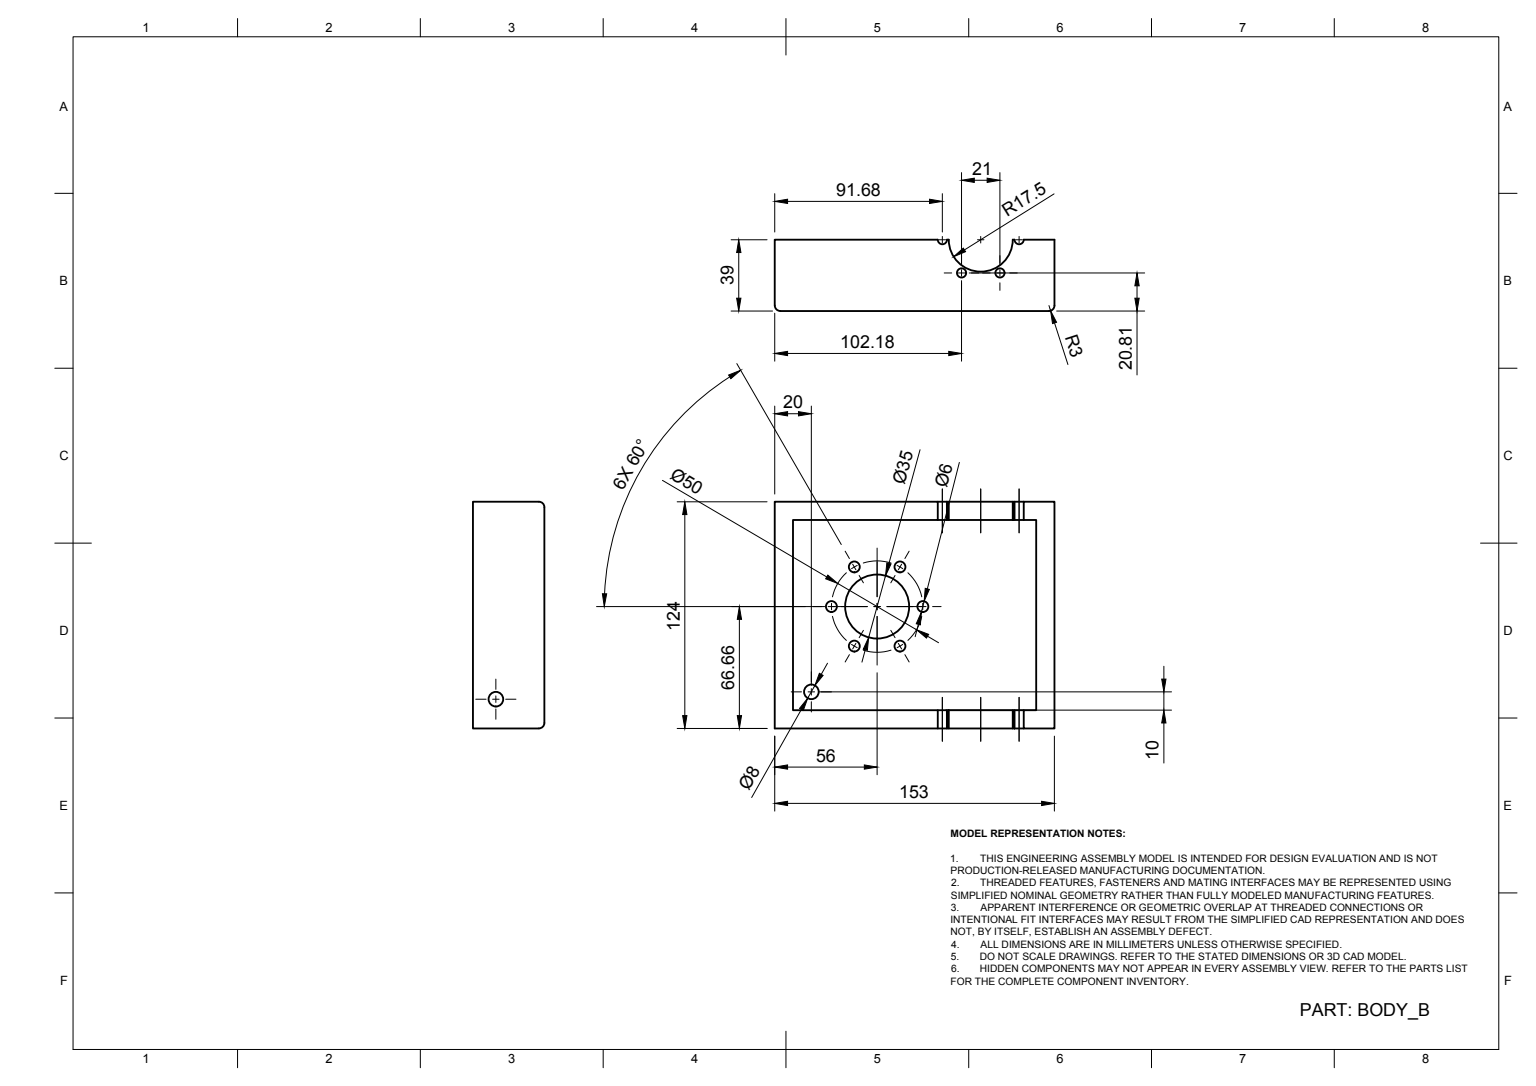
ISO-10303-21;
HEADER;
/* Generated by software containing ST-Developer
 * from STEP Tools, Inc. (www.steptools.com) 
 */

FILE_DESCRIPTION(
/* description */ ('STEP AP214'),
/* implementation_level */ '2;1');

FILE_NAME(
/* name */ 'Body_B.step',
/* time_stamp */ '2026-10-05T13:15:56-07:00',
/* author */ (''),
/* organization */ (''),
/* preprocessor_version */ 'ST-DEVELOPER v20.2',
/* originating_system */ 'Autodesk Translation Framework v15.15.0.0',
/* authorisation */ '');

FILE_SCHEMA (('AUTOMOTIVE_DESIGN { 1 0 10303 214 3 1 1 }'));
ENDSEC;

DATA;
#10=MECHANICAL_DESIGN_GEOMETRIC_PRESENTATION_REPRESENTATION('',(#1349),#37881);
#1325=SHAPE_REPRESENTATION_RELATIONSHIP('SRR','None',#37958,#1337);
#1337=ADVANCED_BREP_SHAPE_REPRESENTATION('',(#1361),#37873);
#1349=STYLED_ITEM('',(#38023),#1361);
#1361=MANIFOLD_SOLID_BREP('Body1',#10823);
#1373=ELLIPSE('',#11682,4.24264068711892,2.99999999999971);
#1374=ELLIPSE('',#11683,4.24264068711757,2.99999999999883);
#1375=ELLIPSE('',#11685,4.24264068711876,2.99999999999963);
#1376=ELLIPSE('',#11687,4.24264068711788,2.99999999999899);
#1407=FACE_BOUND('',#2710,.T.);
#1408=FACE_BOUND('',#2711,.T.);
#1409=FACE_BOUND('',#2714,.T.);
#1410=FACE_BOUND('',#2715,.T.);
#1411=FACE_BOUND('',#2718,.T.);
#1412=FACE_BOUND('',#2720,.T.);
#1413=FACE_BOUND('',#2721,.T.);
#1414=FACE_BOUND('',#2723,.T.);
#1415=FACE_BOUND('',#2725,.T.);
#1416=FACE_BOUND('',#2726,.T.);
#1417=FACE_BOUND('',#2729,.T.);
#1418=FACE_BOUND('',#2730,.T.);
#1419=FACE_BOUND('',#2731,.T.);
#1420=FACE_BOUND('',#2732,.T.);
#1421=FACE_BOUND('',#2733,.T.);
#1422=FACE_BOUND('',#2734,.T.);
#1423=FACE_BOUND('',#2735,.T.);
#1424=FACE_BOUND('',#2736,.T.);
#1425=FACE_BOUND('',#2738,.T.);
#1426=FACE_BOUND('',#2739,.T.);
#1427=FACE_BOUND('',#2740,.T.);
#1428=FACE_BOUND('',#2741,.T.);
#1429=FACE_BOUND('',#2742,.T.);
#1430=FACE_BOUND('',#2743,.T.);
#1431=FACE_BOUND('',#2744,.T.);
#1432=FACE_BOUND('',#2745,.T.);
#1509=PLANE('',#11647);
#1510=PLANE('',#11648);
#1511=PLANE('',#11649);
#1512=PLANE('',#11650);
#1513=PLANE('',#11651);
#1514=PLANE('',#11652);
#1515=PLANE('',#11656);
#1516=PLANE('',#11657);
#1517=PLANE('',#11661);
#1518=PLANE('',#11662);
#1519=PLANE('',#11663);
#1520=PLANE('',#11667);
#1521=PLANE('',#11668);
#1522=PLANE('',#11672);
#1523=PLANE('',#11673);
#1524=PLANE('',#11674);
#2052=FACE_OUTER_BOUND('',#2691,.T.);
#2053=FACE_OUTER_BOUND('',#2692,.T.);
#2054=FACE_OUTER_BOUND('',#2693,.T.);
#2055=FACE_OUTER_BOUND('',#2694,.T.);
#2056=FACE_OUTER_BOUND('',#2695,.T.);
#2057=FACE_OUTER_BOUND('',#2696,.T.);
#2058=FACE_OUTER_BOUND('',#2697,.T.);
#2059=FACE_OUTER_BOUND('',#2698,.T.);
#2060=FACE_OUTER_BOUND('',#2699,.T.);
#2061=FACE_OUTER_BOUND('',#2700,.T.);
#2062=FACE_OUTER_BOUND('',#2701,.T.);
#2063=FACE_OUTER_BOUND('',#2702,.T.);
#2064=FACE_OUTER_BOUND('',#2703,.T.);
#2065=FACE_OUTER_BOUND('',#2704,.T.);
#2066=FACE_OUTER_BOUND('',#2705,.T.);
#2067=FACE_OUTER_BOUND('',#2706,.T.);
#2068=FACE_OUTER_BOUND('',#2707,.T.);
#2069=FACE_OUTER_BOUND('',#2708,.T.);
#2070=FACE_OUTER_BOUND('',#2709,.T.);
#2071=FACE_OUTER_BOUND('',#2712,.T.);
#2072=FACE_OUTER_BOUND('',#2713,.T.);
#2073=FACE_OUTER_BOUND('',#2716,.T.);
#2074=FACE_OUTER_BOUND('',#2717,.T.);
#2075=FACE_OUTER_BOUND('',#2719,.T.);
#2076=FACE_OUTER_BOUND('',#2722,.T.);
#2077=FACE_OUTER_BOUND('',#2724,.T.);
#2078=FACE_OUTER_BOUND('',#2727,.T.);
#2079=FACE_OUTER_BOUND('',#2728,.T.);
#2080=FACE_OUTER_BOUND('',#2737,.T.);
#2081=FACE_OUTER_BOUND('',#2746,.T.);
#2082=FACE_OUTER_BOUND('',#2747,.T.);
#2083=FACE_OUTER_BOUND('',#2748,.T.);
#2084=FACE_OUTER_BOUND('',#2749,.T.);
#2085=FACE_OUTER_BOUND('',#2750,.T.);
#2086=FACE_OUTER_BOUND('',#2751,.T.);
#2087=FACE_OUTER_BOUND('',#2752,.T.);
#2088=FACE_OUTER_BOUND('',#2753,.T.);
#2089=FACE_OUTER_BOUND('',#2754,.T.);
#2090=FACE_OUTER_BOUND('',#2755,.T.);
#2691=EDGE_LOOP('',(#9463,#9464,#9465,#9466));
#2692=EDGE_LOOP('',(#9467,#9468,#9469,#9470));
#2693=EDGE_LOOP('',(#9471,#9472,#9473,#9474));
#2694=EDGE_LOOP('',(#9475,#9476,#9477,#9478));
#2695=EDGE_LOOP('',(#9479,#9480,#9481,#9482));
#2696=EDGE_LOOP('',(#9483,#9484,#9485,#9486));
#2697=EDGE_LOOP('',(#9487,#9488,#9489,#9490));
#2698=EDGE_LOOP('',(#9491,#9492,#9493,#9494));
#2699=EDGE_LOOP('',(#9495,#9496,#9497,#9498));
#2700=EDGE_LOOP('',(#9499,#9500,#9501,#9502));
#2701=EDGE_LOOP('',(#9503,#9504,#9505,#9506));
#2702=EDGE_LOOP('',(#9507,#9508,#9509,#9510));
#2703=EDGE_LOOP('',(#9511,#9512,#9513,#9514));
#2704=EDGE_LOOP('',(#9515,#9516,#9517,#9518,#9519,#9520,#9521,#9522));
#2705=EDGE_LOOP('',(#9523,#9524,#9525,#9526));
#2706=EDGE_LOOP('',(#9527,#9528,#9529,#9530));
#2707=EDGE_LOOP('',(#9531,#9532,#9533,#9534));
#2708=EDGE_LOOP('',(#9535,#9536,#9537,#9538));
#2709=EDGE_LOOP('',(#9539,#9540,#9541,#9542,#9543,#9544,#9545,#9546,#9547,
#9548));
#2710=EDGE_LOOP('',(#9549));
#2711=EDGE_LOOP('',(#9550));
#2712=EDGE_LOOP('',(#9551,#9552,#9553,#9554,#9555,#9556,#9557,#9558));
#2713=EDGE_LOOP('',(#9559,#9560,#9561,#9562,#9563,#9564,#9565,#9566,#9567,
#9568));
#2714=EDGE_LOOP('',(#9569));
#2715=EDGE_LOOP('',(#9570));
#2716=EDGE_LOOP('',(#9571,#9572,#9573,#9574));
#2717=EDGE_LOOP('',(#9575,#9576,#9577,#9578));
#2718=EDGE_LOOP('',(#9579));
#2719=EDGE_LOOP('',(#9580,#9581,#9582,#9583,#9584,#9585,#9586,#9587,#9588,
#9589));
#2720=EDGE_LOOP('',(#9590));
#2721=EDGE_LOOP('',(#9591));
#2722=EDGE_LOOP('',(#9592,#9593,#9594,#9595));
#2723=EDGE_LOOP('',(#9596));
#2724=EDGE_LOOP('',(#9597,#9598,#9599,#9600,#9601,#9602,#9603,#9604,#9605,
#9606));
#2725=EDGE_LOOP('',(#9607));
#2726=EDGE_LOOP('',(#9608));
#2727=EDGE_LOOP('',(#9609,#9610,#9611,#9612));
#2728=EDGE_LOOP('',(#9613,#9614,#9615,#9616));
#2729=EDGE_LOOP('',(#9617));
#2730=EDGE_LOOP('',(#9618));
#2731=EDGE_LOOP('',(#9619));
#2732=EDGE_LOOP('',(#9620));
#2733=EDGE_LOOP('',(#9621));
#2734=EDGE_LOOP('',(#9622));
#2735=EDGE_LOOP('',(#9623));
#2736=EDGE_LOOP('',(#9624));
#2737=EDGE_LOOP('',(#9625,#9626,#9627,#9628));
#2738=EDGE_LOOP('',(#9629));
#2739=EDGE_LOOP('',(#9630));
#2740=EDGE_LOOP('',(#9631));
#2741=EDGE_LOOP('',(#9632));
#2742=EDGE_LOOP('',(#9633));
#2743=EDGE_LOOP('',(#9634));
#2744=EDGE_LOOP('',(#9635));
#2745=EDGE_LOOP('',(#9636));
#2746=EDGE_LOOP('',(#9637,#9638,#9639,#9640));
#2747=EDGE_LOOP('',(#9641,#9642,#9643,#9644));
#2748=EDGE_LOOP('',(#9645,#9646,#9647,#9648));
#2749=EDGE_LOOP('',(#9649,#9650,#9651,#9652));
#2750=EDGE_LOOP('',(#9653,#9654,#9655,#9656));
#2751=EDGE_LOOP('',(#9657,#9658,#9659,#9660));
#2752=EDGE_LOOP('',(#9661,#9662,#9663,#9664));
#2753=EDGE_LOOP('',(#9665,#9666,#9667,#9668));
#2754=EDGE_LOOP('',(#9669,#9670,#9671,#9672));
#2755=EDGE_LOOP('',(#9673,#9674,#9675,#9676));
#3001=LINE('',#37226,#3302);
#3002=LINE('',#37232,#3303);
#3003=LINE('',#37238,#3304);
#3004=LINE('',#37244,#3305);
#3005=LINE('',#37250,#3306);
#3006=LINE('',#37256,#3307);
#3007=LINE('',#37262,#3308);
#3008=LINE('',#37268,#3309);
#3009=LINE('',#37274,#3310);
#3010=LINE('',#37280,#3311);
#3011=LINE('',#37286,#3312);
#3012=LINE('',#37292,#3313);
#3013=LINE('',#37298,#3314);
#3014=LINE('',#37303,#3315);
#3015=LINE('',#37305,#3316);
#3016=LINE('',#37307,#3317);
#3017=LINE('',#37309,#3318);
#3018=LINE('',#37311,#3319);
#3019=LINE('',#37313,#3320);
#3020=LINE('',#37315,#3321);
#3021=LINE('',#37316,#3322);
#3022=LINE('',#37320,#3323);
#3023=LINE('',#37322,#3324);
#3024=LINE('',#37324,#3325);
#3025=LINE('',#37325,#3326);
#3026=LINE('',#37329,#3327);
#3027=LINE('',#37331,#3328);
#3028=LINE('',#37333,#3329);
#3029=LINE('',#37334,#3330);
#3030=LINE('',#37338,#3331);
#3031=LINE('',#37340,#3332);
#3032=LINE('',#37342,#3333);
#3033=LINE('',#37343,#3334);
#3034=LINE('',#37347,#3335);
#3035=LINE('',#37349,#3336);
#3036=LINE('',#37351,#3337);
#3037=LINE('',#37352,#3338);
#3038=LINE('',#37355,#3339);
#3039=LINE('',#37361,#3340);
#3040=LINE('',#37363,#3341);
#3041=LINE('',#37364,#3342);
#3042=LINE('',#37367,#3343);
#3043=LINE('',#37369,#3344);
#3044=LINE('',#37371,#3345);
#3045=LINE('',#37373,#3346);
#3046=LINE('',#37375,#3347);
#3047=LINE('',#37377,#3348);
#3048=LINE('',#37378,#3349);
#3049=LINE('',#37381,#3350);
#3050=LINE('',#37386,#3351);
#3051=LINE('',#37387,#3352);
#3052=LINE('',#37389,#3353);
#3053=LINE('',#37391,#3354);
#3054=LINE('',#37395,#3355);
#3055=LINE('',#37397,#3356);
#3056=LINE('',#37398,#3357);
#3057=LINE('',#37403,#3358);
#3058=LINE('',#37404,#3359);
#3059=LINE('',#37410,#3360);
#3060=LINE('',#37411,#3361);
#3061=LINE('',#37413,#3362);
#3062=LINE('',#37418,#3363);
#3063=LINE('',#37420,#3364);
#3064=LINE('',#37422,#3365);
#3065=LINE('',#37423,#3366);
#3302=VECTOR('',#13312,4.);
#3303=VECTOR('',#13319,4.);
#3304=VECTOR('',#13326,2.5);
#3305=VECTOR('',#13333,2.5);
#3306=VECTOR('',#13340,2.5);
#3307=VECTOR('',#13347,2.5);
#3308=VECTOR('',#13354,3.);
#3309=VECTOR('',#13361,2.99999999999999);
#3310=VECTOR('',#13368,3.);
#3311=VECTOR('',#13375,3.);
#3312=VECTOR('',#13382,3.);
#3313=VECTOR('',#13389,3.);
#3314=VECTOR('',#13396,17.5);
#3315=VECTOR('',#13401,1000.);
#3316=VECTOR('',#13402,1000.);
#3317=VECTOR('',#13403,1000.);
#3318=VECTOR('',#13404,1000.);
#3319=VECTOR('',#13405,1000.);
#3320=VECTOR('',#13406,1000.);
#3321=VECTOR('',#13407,1000.);
#3322=VECTOR('',#13408,1000.);
#3323=VECTOR('',#13411,1000.);
#3324=VECTOR('',#13412,1000.);
#3325=VECTOR('',#13413,1000.);
#3326=VECTOR('',#13414,1000.);
#3327=VECTOR('',#13417,1000.);
#3328=VECTOR('',#13418,1000.);
#3329=VECTOR('',#13419,1000.);
#3330=VECTOR('',#13420,1000.);
#3331=VECTOR('',#13423,1000.);
#3332=VECTOR('',#13424,1000.);
#3333=VECTOR('',#13425,1000.);
#3334=VECTOR('',#13426,1000.);
#3335=VECTOR('',#13429,1000.);
#3336=VECTOR('',#13430,1000.);
#3337=VECTOR('',#13431,1000.);
#3338=VECTOR('',#13432,1000.);
#3339=VECTOR('',#13435,1000.);
#3340=VECTOR('',#13442,1000.);
#3341=VECTOR('',#13443,1000.);
#3342=VECTOR('',#13444,1000.);
#3343=VECTOR('',#13447,1000.);
#3344=VECTOR('',#13448,1000.);
#3345=VECTOR('',#13449,1000.);
#3346=VECTOR('',#13450,1000.);
#3347=VECTOR('',#13451,1000.);
#3348=VECTOR('',#13452,1000.);
#3349=VECTOR('',#13453,1000.);
#3350=VECTOR('',#13456,1000.);
#3351=VECTOR('',#13463,1000.);
#3352=VECTOR('',#13464,1000.);
#3353=VECTOR('',#13467,1000.);
#3354=VECTOR('',#13470,1000.);
#3355=VECTOR('',#13475,1000.);
#3356=VECTOR('',#13476,1000.);
#3357=VECTOR('',#13477,1000.);
#3358=VECTOR('',#13484,1000.);
#3359=VECTOR('',#13485,1000.);
#3360=VECTOR('',#13494,1000.);
#3361=VECTOR('',#13495,1000.);
#3362=VECTOR('',#13498,1000.);
#3363=VECTOR('',#13503,1000.);
#3364=VECTOR('',#13504,1000.);
#3365=VECTOR('',#13505,1000.);
#3366=VECTOR('',#13506,1000.);
#3890=CIRCLE('',#11609,4.);
#3891=CIRCLE('',#11610,4.);
#3892=CIRCLE('',#11612,4.);
#3893=CIRCLE('',#11613,4.);
#3894=CIRCLE('',#11615,2.5);
#3895=CIRCLE('',#11616,2.5);
#3896=CIRCLE('',#11618,2.5);
#3897=CIRCLE('',#11619,2.5);
#3898=CIRCLE('',#11621,2.5);
#3899=CIRCLE('',#11622,2.5);
#3900=CIRCLE('',#11624,2.5);
#3901=CIRCLE('',#11625,2.5);
#3902=CIRCLE('',#11627,3.);
#3903=CIRCLE('',#11628,3.);
#3904=CIRCLE('',#11630,2.99999999999999);
#3905=CIRCLE('',#11631,2.99999999999999);
#3906=CIRCLE('',#11633,3.);
#3907=CIRCLE('',#11634,3.);
#3908=CIRCLE('',#11636,3.);
#3909=CIRCLE('',#11637,3.);
#3910=CIRCLE('',#11639,3.);
#3911=CIRCLE('',#11640,3.);
#3912=CIRCLE('',#11642,3.);
#3913=CIRCLE('',#11643,3.);
#3914=CIRCLE('',#11645,17.5);
#3915=CIRCLE('',#11646,17.5);
#3916=CIRCLE('',#11653,2.5);
#3917=CIRCLE('',#11654,17.5);
#3918=CIRCLE('',#11655,2.50000000000001);
#3919=CIRCLE('',#11658,2.50000000000001);
#3920=CIRCLE('',#11659,17.5);
#3921=CIRCLE('',#11660,2.5);
#3922=CIRCLE('',#11664,2.5);
#3923=CIRCLE('',#11665,2.50000000000001);
#3924=CIRCLE('',#11666,17.5);
#3925=CIRCLE('',#11669,2.5);
#3926=CIRCLE('',#11670,17.5);
#3927=CIRCLE('',#11671,2.50000000000001);
#4894=VERTEX_POINT('',#37223);
#4895=VERTEX_POINT('',#37225);
#4896=VERTEX_POINT('',#37229);
#4897=VERTEX_POINT('',#37231);
#4898=VERTEX_POINT('',#37235);
#4899=VERTEX_POINT('',#37237);
#4900=VERTEX_POINT('',#37241);
#4901=VERTEX_POINT('',#37243);
#4902=VERTEX_POINT('',#37247);
#4903=VERTEX_POINT('',#37249);
#4904=VERTEX_POINT('',#37253);
#4905=VERTEX_POINT('',#37255);
#4906=VERTEX_POINT('',#37259);
#4907=VERTEX_POINT('',#37261);
#4908=VERTEX_POINT('',#37265);
#4909=VERTEX_POINT('',#37267);
#4910=VERTEX_POINT('',#37271);
#4911=VERTEX_POINT('',#37273);
#4912=VERTEX_POINT('',#37277);
#4913=VERTEX_POINT('',#37279);
#4914=VERTEX_POINT('',#37283);
#4915=VERTEX_POINT('',#37285);
#4916=VERTEX_POINT('',#37289);
#4917=VERTEX_POINT('',#37291);
#4918=VERTEX_POINT('',#37295);
#4919=VERTEX_POINT('',#37297);
#4920=VERTEX_POINT('',#37301);
#4921=VERTEX_POINT('',#37302);
#4922=VERTEX_POINT('',#37304);
#4923=VERTEX_POINT('',#37306);
#4924=VERTEX_POINT('',#37308);
#4925=VERTEX_POINT('',#37310);
#4926=VERTEX_POINT('',#37312);
#4927=VERTEX_POINT('',#37314);
#4928=VERTEX_POINT('',#37318);
#4929=VERTEX_POINT('',#37319);
#4930=VERTEX_POINT('',#37321);
#4931=VERTEX_POINT('',#37323);
#4932=VERTEX_POINT('',#37327);
#4933=VERTEX_POINT('',#37328);
#4934=VERTEX_POINT('',#37330);
#4935=VERTEX_POINT('',#37332);
#4936=VERTEX_POINT('',#37336);
#4937=VERTEX_POINT('',#37337);
#4938=VERTEX_POINT('',#37339);
#4939=VERTEX_POINT('',#37341);
#4940=VERTEX_POINT('',#37345);
#4941=VERTEX_POINT('',#37346);
#4942=VERTEX_POINT('',#37348);
#4943=VERTEX_POINT('',#37350);
#4944=VERTEX_POINT('',#37354);
#4945=VERTEX_POINT('',#37358);
#4946=VERTEX_POINT('',#37360);
#4947=VERTEX_POINT('',#37362);
#4948=VERTEX_POINT('',#37366);
#4949=VERTEX_POINT('',#37368);
#4950=VERTEX_POINT('',#37370);
#4951=VERTEX_POINT('',#37372);
#4952=VERTEX_POINT('',#37374);
#4953=VERTEX_POINT('',#37376);
#4954=VERTEX_POINT('',#37380);
#4955=VERTEX_POINT('',#37385);
#4956=VERTEX_POINT('',#37394);
#4957=VERTEX_POINT('',#37396);
#4958=VERTEX_POINT('',#37402);
#4959=VERTEX_POINT('',#37409);
#4960=VERTEX_POINT('',#37416);
#4961=VERTEX_POINT('',#37417);
#4962=VERTEX_POINT('',#37419);
#4963=VERTEX_POINT('',#37421);
#6442=EDGE_CURVE('',#4894,#4894,#3890,.T.);
#6443=EDGE_CURVE('',#4894,#4895,#3001,.T.);
#6444=EDGE_CURVE('',#4895,#4895,#3891,.T.);
#6445=EDGE_CURVE('',#4896,#4896,#3892,.T.);
#6446=EDGE_CURVE('',#4896,#4897,#3002,.T.);
#6447=EDGE_CURVE('',#4897,#4897,#3893,.T.);
#6448=EDGE_CURVE('',#4898,#4898,#3894,.T.);
#6449=EDGE_CURVE('',#4898,#4899,#3003,.T.);
#6450=EDGE_CURVE('',#4899,#4899,#3895,.T.);
#6451=EDGE_CURVE('',#4900,#4900,#3896,.T.);
#6452=EDGE_CURVE('',#4900,#4901,#3004,.T.);
#6453=EDGE_CURVE('',#4901,#4901,#3897,.T.);
#6454=EDGE_CURVE('',#4902,#4902,#3898,.T.);
#6455=EDGE_CURVE('',#4902,#4903,#3005,.T.);
#6456=EDGE_CURVE('',#4903,#4903,#3899,.T.);
#6457=EDGE_CURVE('',#4904,#4904,#3900,.T.);
#6458=EDGE_CURVE('',#4904,#4905,#3006,.T.);
#6459=EDGE_CURVE('',#4905,#4905,#3901,.T.);
#6460=EDGE_CURVE('',#4906,#4906,#3902,.T.);
#6461=EDGE_CURVE('',#4906,#4907,#3007,.T.);
#6462=EDGE_CURVE('',#4907,#4907,#3903,.T.);
#6463=EDGE_CURVE('',#4908,#4908,#3904,.T.);
#6464=EDGE_CURVE('',#4908,#4909,#3008,.T.);
#6465=EDGE_CURVE('',#4909,#4909,#3905,.T.);
#6466=EDGE_CURVE('',#4910,#4910,#3906,.T.);
#6467=EDGE_CURVE('',#4910,#4911,#3009,.T.);
#6468=EDGE_CURVE('',#4911,#4911,#3907,.T.);
#6469=EDGE_CURVE('',#4912,#4912,#3908,.T.);
#6470=EDGE_CURVE('',#4912,#4913,#3010,.T.);
#6471=EDGE_CURVE('',#4913,#4913,#3909,.T.);
#6472=EDGE_CURVE('',#4914,#4914,#3910,.T.);
#6473=EDGE_CURVE('',#4914,#4915,#3011,.T.);
#6474=EDGE_CURVE('',#4915,#4915,#3911,.T.);
#6475=EDGE_CURVE('',#4916,#4916,#3912,.T.);
#6476=EDGE_CURVE('',#4916,#4917,#3012,.T.);
#6477=EDGE_CURVE('',#4917,#4917,#3913,.T.);
#6478=EDGE_CURVE('',#4918,#4918,#3914,.T.);
#6479=EDGE_CURVE('',#4918,#4919,#3013,.T.);
#6480=EDGE_CURVE('',#4919,#4919,#3915,.T.);
#6481=EDGE_CURVE('',#4920,#4921,#3014,.T.);
#6482=EDGE_CURVE('',#4922,#4921,#3015,.T.);
#6483=EDGE_CURVE('',#4923,#4922,#3016,.T.);
#6484=EDGE_CURVE('',#4924,#4923,#3017,.T.);
#6485=EDGE_CURVE('',#4924,#4925,#3018,.T.);
#6486=EDGE_CURVE('',#4925,#4926,#3019,.T.);
#6487=EDGE_CURVE('',#4926,#4927,#3020,.T.);
#6488=EDGE_CURVE('',#4927,#4920,#3021,.T.);
#6489=EDGE_CURVE('',#4928,#4929,#3022,.T.);
#6490=EDGE_CURVE('',#4930,#4929,#3023,.T.);
#6491=EDGE_CURVE('',#4930,#4931,#3024,.T.);
#6492=EDGE_CURVE('',#4931,#4928,#3025,.T.);
#6493=EDGE_CURVE('',#4932,#4933,#3026,.T.);
#6494=EDGE_CURVE('',#4933,#4934,#3027,.T.);
#6495=EDGE_CURVE('',#4934,#4935,#3028,.T.);
#6496=EDGE_CURVE('',#4932,#4935,#3029,.T.);
#6497=EDGE_CURVE('',#4936,#4937,#3030,.T.);
#6498=EDGE_CURVE('',#4938,#4937,#3031,.T.);
#6499=EDGE_CURVE('',#4938,#4939,#3032,.T.);
#6500=EDGE_CURVE('',#4939,#4936,#3033,.T.);
#6501=EDGE_CURVE('',#4940,#4941,#3034,.T.);
#6502=EDGE_CURVE('',#4941,#4942,#3035,.T.);
#6503=EDGE_CURVE('',#4942,#4943,#3036,.T.);
#6504=EDGE_CURVE('',#4940,#4943,#3037,.T.);
#6505=EDGE_CURVE('',#4944,#4926,#3038,.T.);
#6506=EDGE_CURVE('',#4925,#4928,#3916,.T.);
#6507=EDGE_CURVE('',#4931,#4934,#3917,.T.);
#6508=EDGE_CURVE('',#4933,#4945,#3918,.T.);
#6509=EDGE_CURVE('',#4946,#4945,#3039,.T.);
#6510=EDGE_CURVE('',#4947,#4946,#3040,.T.);
#6511=EDGE_CURVE('',#4944,#4947,#3041,.T.);
#6512=EDGE_CURVE('',#4945,#4948,#3042,.T.);
#6513=EDGE_CURVE('',#4949,#4948,#3043,.T.);
#6514=EDGE_CURVE('',#4950,#4949,#3044,.T.);
#6515=EDGE_CURVE('',#4951,#4950,#3045,.T.);
#6516=EDGE_CURVE('',#4951,#4952,#3046,.T.);
#6517=EDGE_CURVE('',#4952,#4953,#3047,.T.);
#6518=EDGE_CURVE('',#4953,#4946,#3048,.T.);
#6519=EDGE_CURVE('',#4954,#4953,#3049,.T.);
#6520=EDGE_CURVE('',#4936,#4952,#3919,.T.);
#6521=EDGE_CURVE('',#4942,#4939,#3920,.T.);
#6522=EDGE_CURVE('',#4920,#4941,#3921,.T.);
#6523=EDGE_CURVE('',#4955,#4927,#3050,.T.);
#6524=EDGE_CURVE('',#4954,#4955,#3051,.T.);
#6525=EDGE_CURVE('',#4947,#4954,#3052,.T.);
#6526=EDGE_CURVE('',#4955,#4944,#3053,.T.);
#6527=EDGE_CURVE('',#4929,#4924,#3922,.T.);
#6528=EDGE_CURVE('',#4956,#4923,#3054,.T.);
#6529=EDGE_CURVE('',#4957,#4956,#3055,.T.);
#6530=EDGE_CURVE('',#4957,#4949,#3056,.T.);
#6531=EDGE_CURVE('',#4948,#4932,#3923,.T.);
#6532=EDGE_CURVE('',#4935,#4930,#3924,.T.);
#6533=EDGE_CURVE('',#4958,#4922,#3057,.T.);
#6534=EDGE_CURVE('',#4956,#4958,#3058,.T.);
#6535=EDGE_CURVE('',#4921,#4940,#3925,.T.);
#6536=EDGE_CURVE('',#4943,#4938,#3926,.T.);
#6537=EDGE_CURVE('',#4937,#4951,#3927,.T.);
#6538=EDGE_CURVE('',#4959,#4950,#3059,.T.);
#6539=EDGE_CURVE('',#4958,#4959,#3060,.T.);
#6540=EDGE_CURVE('',#4959,#4957,#3061,.T.);
#6541=EDGE_CURVE('',#4960,#4961,#3062,.T.);
#6542=EDGE_CURVE('',#4962,#4960,#3063,.T.);
#6543=EDGE_CURVE('',#4963,#4962,#3064,.T.);
#6544=EDGE_CURVE('',#4961,#4963,#3065,.T.);
#6545=EDGE_CURVE('',#4947,#4962,#1373,.T.);
#6546=EDGE_CURVE('',#4960,#4944,#1374,.T.);
#6547=EDGE_CURVE('',#4961,#4955,#1375,.T.);
#6548=EDGE_CURVE('',#4954,#4963,#1376,.T.);
#9463=ORIENTED_EDGE('',*,*,#6442,.F.);
#9464=ORIENTED_EDGE('',*,*,#6443,.T.);
#9465=ORIENTED_EDGE('',*,*,#6444,.T.);
#9466=ORIENTED_EDGE('',*,*,#6443,.F.);
#9467=ORIENTED_EDGE('',*,*,#6445,.F.);
#9468=ORIENTED_EDGE('',*,*,#6446,.T.);
#9469=ORIENTED_EDGE('',*,*,#6447,.T.);
#9470=ORIENTED_EDGE('',*,*,#6446,.F.);
#9471=ORIENTED_EDGE('',*,*,#6448,.F.);
#9472=ORIENTED_EDGE('',*,*,#6449,.T.);
#9473=ORIENTED_EDGE('',*,*,#6450,.F.);
#9474=ORIENTED_EDGE('',*,*,#6449,.F.);
#9475=ORIENTED_EDGE('',*,*,#6451,.F.);
#9476=ORIENTED_EDGE('',*,*,#6452,.T.);
#9477=ORIENTED_EDGE('',*,*,#6453,.F.);
#9478=ORIENTED_EDGE('',*,*,#6452,.F.);
#9479=ORIENTED_EDGE('',*,*,#6454,.T.);
#9480=ORIENTED_EDGE('',*,*,#6455,.T.);
#9481=ORIENTED_EDGE('',*,*,#6456,.F.);
#9482=ORIENTED_EDGE('',*,*,#6455,.F.);
#9483=ORIENTED_EDGE('',*,*,#6457,.T.);
#9484=ORIENTED_EDGE('',*,*,#6458,.T.);
#9485=ORIENTED_EDGE('',*,*,#6459,.F.);
#9486=ORIENTED_EDGE('',*,*,#6458,.F.);
#9487=ORIENTED_EDGE('',*,*,#6460,.T.);
#9488=ORIENTED_EDGE('',*,*,#6461,.T.);
#9489=ORIENTED_EDGE('',*,*,#6462,.F.);
#9490=ORIENTED_EDGE('',*,*,#6461,.F.);
#9491=ORIENTED_EDGE('',*,*,#6463,.T.);
#9492=ORIENTED_EDGE('',*,*,#6464,.T.);
#9493=ORIENTED_EDGE('',*,*,#6465,.F.);
#9494=ORIENTED_EDGE('',*,*,#6464,.F.);
#9495=ORIENTED_EDGE('',*,*,#6466,.T.);
#9496=ORIENTED_EDGE('',*,*,#6467,.T.);
#9497=ORIENTED_EDGE('',*,*,#6468,.F.);
#9498=ORIENTED_EDGE('',*,*,#6467,.F.);
#9499=ORIENTED_EDGE('',*,*,#6469,.T.);
#9500=ORIENTED_EDGE('',*,*,#6470,.T.);
#9501=ORIENTED_EDGE('',*,*,#6471,.F.);
#9502=ORIENTED_EDGE('',*,*,#6470,.F.);
#9503=ORIENTED_EDGE('',*,*,#6472,.T.);
#9504=ORIENTED_EDGE('',*,*,#6473,.T.);
#9505=ORIENTED_EDGE('',*,*,#6474,.F.);
#9506=ORIENTED_EDGE('',*,*,#6473,.F.);
#9507=ORIENTED_EDGE('',*,*,#6475,.T.);
#9508=ORIENTED_EDGE('',*,*,#6476,.T.);
#9509=ORIENTED_EDGE('',*,*,#6477,.F.);
#9510=ORIENTED_EDGE('',*,*,#6476,.F.);
#9511=ORIENTED_EDGE('',*,*,#6478,.T.);
#9512=ORIENTED_EDGE('',*,*,#6479,.T.);
#9513=ORIENTED_EDGE('',*,*,#6480,.F.);
#9514=ORIENTED_EDGE('',*,*,#6479,.F.);
#9515=ORIENTED_EDGE('',*,*,#6481,.T.);
#9516=ORIENTED_EDGE('',*,*,#6482,.F.);
#9517=ORIENTED_EDGE('',*,*,#6483,.F.);
#9518=ORIENTED_EDGE('',*,*,#6484,.F.);
#9519=ORIENTED_EDGE('',*,*,#6485,.T.);
#9520=ORIENTED_EDGE('',*,*,#6486,.T.);
#9521=ORIENTED_EDGE('',*,*,#6487,.T.);
#9522=ORIENTED_EDGE('',*,*,#6488,.T.);
#9523=ORIENTED_EDGE('',*,*,#6489,.T.);
#9524=ORIENTED_EDGE('',*,*,#6490,.F.);
#9525=ORIENTED_EDGE('',*,*,#6491,.T.);
#9526=ORIENTED_EDGE('',*,*,#6492,.T.);
#9527=ORIENTED_EDGE('',*,*,#6493,.T.);
#9528=ORIENTED_EDGE('',*,*,#6494,.T.);
#9529=ORIENTED_EDGE('',*,*,#6495,.T.);
#9530=ORIENTED_EDGE('',*,*,#6496,.F.);
#9531=ORIENTED_EDGE('',*,*,#6497,.T.);
#9532=ORIENTED_EDGE('',*,*,#6498,.F.);
#9533=ORIENTED_EDGE('',*,*,#6499,.T.);
#9534=ORIENTED_EDGE('',*,*,#6500,.T.);
#9535=ORIENTED_EDGE('',*,*,#6501,.T.);
#9536=ORIENTED_EDGE('',*,*,#6502,.T.);
#9537=ORIENTED_EDGE('',*,*,#6503,.T.);
#9538=ORIENTED_EDGE('',*,*,#6504,.F.);
#9539=ORIENTED_EDGE('',*,*,#6505,.T.);
#9540=ORIENTED_EDGE('',*,*,#6486,.F.);
#9541=ORIENTED_EDGE('',*,*,#6506,.T.);
#9542=ORIENTED_EDGE('',*,*,#6492,.F.);
#9543=ORIENTED_EDGE('',*,*,#6507,.T.);
#9544=ORIENTED_EDGE('',*,*,#6494,.F.);
#9545=ORIENTED_EDGE('',*,*,#6508,.T.);
#9546=ORIENTED_EDGE('',*,*,#6509,.F.);
#9547=ORIENTED_EDGE('',*,*,#6510,.F.);
#9548=ORIENTED_EDGE('',*,*,#6511,.F.);
#9549=ORIENTED_EDGE('',*,*,#6453,.T.);
#9550=ORIENTED_EDGE('',*,*,#6450,.T.);
#9551=ORIENTED_EDGE('',*,*,#6512,.T.);
#9552=ORIENTED_EDGE('',*,*,#6513,.F.);
#9553=ORIENTED_EDGE('',*,*,#6514,.F.);
#9554=ORIENTED_EDGE('',*,*,#6515,.F.);
#9555=ORIENTED_EDGE('',*,*,#6516,.T.);
#9556=ORIENTED_EDGE('',*,*,#6517,.T.);
#9557=ORIENTED_EDGE('',*,*,#6518,.T.);
#9558=ORIENTED_EDGE('',*,*,#6509,.T.);
#9559=ORIENTED_EDGE('',*,*,#6519,.T.);
#9560=ORIENTED_EDGE('',*,*,#6517,.F.);
#9561=ORIENTED_EDGE('',*,*,#6520,.F.);
#9562=ORIENTED_EDGE('',*,*,#6500,.F.);
#9563=ORIENTED_EDGE('',*,*,#6521,.F.);
#9564=ORIENTED_EDGE('',*,*,#6502,.F.);
#9565=ORIENTED_EDGE('',*,*,#6522,.F.);
#9566=ORIENTED_EDGE('',*,*,#6488,.F.);
#9567=ORIENTED_EDGE('',*,*,#6523,.F.);
#9568=ORIENTED_EDGE('',*,*,#6524,.F.);
#9569=ORIENTED_EDGE('',*,*,#6454,.F.);
#9570=ORIENTED_EDGE('',*,*,#6457,.F.);
#9571=ORIENTED_EDGE('',*,*,#6510,.T.);
#9572=ORIENTED_EDGE('',*,*,#6518,.F.);
#9573=ORIENTED_EDGE('',*,*,#6519,.F.);
#9574=ORIENTED_EDGE('',*,*,#6525,.F.);
#9575=ORIENTED_EDGE('',*,*,#6523,.T.);
#9576=ORIENTED_EDGE('',*,*,#6487,.F.);
#9577=ORIENTED_EDGE('',*,*,#6505,.F.);
#9578=ORIENTED_EDGE('',*,*,#6526,.F.);
#9579=ORIENTED_EDGE('',*,*,#6444,.F.);
#9580=ORIENTED_EDGE('',*,*,#6527,.T.);
#9581=ORIENTED_EDGE('',*,*,#6484,.T.);
#9582=ORIENTED_EDGE('',*,*,#6528,.F.);
#9583=ORIENTED_EDGE('',*,*,#6529,.F.);
#9584=ORIENTED_EDGE('',*,*,#6530,.T.);
#9585=ORIENTED_EDGE('',*,*,#6513,.T.);
#9586=ORIENTED_EDGE('',*,*,#6531,.T.);
#9587=ORIENTED_EDGE('',*,*,#6496,.T.);
#9588=ORIENTED_EDGE('',*,*,#6532,.T.);
#9589=ORIENTED_EDGE('',*,*,#6490,.T.);
#9590=ORIENTED_EDGE('',*,*,#6448,.T.);
#9591=ORIENTED_EDGE('',*,*,#6451,.T.);
#9592=ORIENTED_EDGE('',*,*,#6483,.T.);
#9593=ORIENTED_EDGE('',*,*,#6533,.F.);
#9594=ORIENTED_EDGE('',*,*,#6534,.F.);
#9595=ORIENTED_EDGE('',*,*,#6528,.T.);
#9596=ORIENTED_EDGE('',*,*,#6442,.T.);
#9597=ORIENTED_EDGE('',*,*,#6535,.T.);
#9598=ORIENTED_EDGE('',*,*,#6504,.T.);
#9599=ORIENTED_EDGE('',*,*,#6536,.T.);
#9600=ORIENTED_EDGE('',*,*,#6498,.T.);
#9601=ORIENTED_EDGE('',*,*,#6537,.T.);
#9602=ORIENTED_EDGE('',*,*,#6515,.T.);
#9603=ORIENTED_EDGE('',*,*,#6538,.F.);
#9604=ORIENTED_EDGE('',*,*,#6539,.F.);
#9605=ORIENTED_EDGE('',*,*,#6533,.T.);
#9606=ORIENTED_EDGE('',*,*,#6482,.T.);
#9607=ORIENTED_EDGE('',*,*,#6456,.T.);
#9608=ORIENTED_EDGE('',*,*,#6459,.T.);
#9609=ORIENTED_EDGE('',*,*,#6514,.T.);
#9610=ORIENTED_EDGE('',*,*,#6530,.F.);
#9611=ORIENTED_EDGE('',*,*,#6540,.F.);
#9612=ORIENTED_EDGE('',*,*,#6538,.T.);
#9613=ORIENTED_EDGE('',*,*,#6529,.T.);
#9614=ORIENTED_EDGE('',*,*,#6534,.T.);
#9615=ORIENTED_EDGE('',*,*,#6539,.T.);
#9616=ORIENTED_EDGE('',*,*,#6540,.T.);
#9617=ORIENTED_EDGE('',*,*,#6445,.T.);
#9618=ORIENTED_EDGE('',*,*,#6460,.F.);
#9619=ORIENTED_EDGE('',*,*,#6463,.F.);
#9620=ORIENTED_EDGE('',*,*,#6466,.F.);
#9621=ORIENTED_EDGE('',*,*,#6469,.F.);
#9622=ORIENTED_EDGE('',*,*,#6472,.F.);
#9623=ORIENTED_EDGE('',*,*,#6475,.F.);
#9624=ORIENTED_EDGE('',*,*,#6478,.F.);
#9625=ORIENTED_EDGE('',*,*,#6541,.F.);
#9626=ORIENTED_EDGE('',*,*,#6542,.F.);
#9627=ORIENTED_EDGE('',*,*,#6543,.F.);
#9628=ORIENTED_EDGE('',*,*,#6544,.F.);
#9629=ORIENTED_EDGE('',*,*,#6462,.T.);
#9630=ORIENTED_EDGE('',*,*,#6465,.T.);
#9631=ORIENTED_EDGE('',*,*,#6468,.T.);
#9632=ORIENTED_EDGE('',*,*,#6471,.T.);
#9633=ORIENTED_EDGE('',*,*,#6474,.T.);
#9634=ORIENTED_EDGE('',*,*,#6477,.T.);
#9635=ORIENTED_EDGE('',*,*,#6480,.T.);
#9636=ORIENTED_EDGE('',*,*,#6447,.F.);
#9637=ORIENTED_EDGE('',*,*,#6503,.F.);
#9638=ORIENTED_EDGE('',*,*,#6521,.T.);
#9639=ORIENTED_EDGE('',*,*,#6499,.F.);
#9640=ORIENTED_EDGE('',*,*,#6536,.F.);
#9641=ORIENTED_EDGE('',*,*,#6497,.F.);
#9642=ORIENTED_EDGE('',*,*,#6520,.T.);
#9643=ORIENTED_EDGE('',*,*,#6516,.F.);
#9644=ORIENTED_EDGE('',*,*,#6537,.F.);
#9645=ORIENTED_EDGE('',*,*,#6481,.F.);
#9646=ORIENTED_EDGE('',*,*,#6522,.T.);
#9647=ORIENTED_EDGE('',*,*,#6501,.F.);
#9648=ORIENTED_EDGE('',*,*,#6535,.F.);
#9649=ORIENTED_EDGE('',*,*,#6491,.F.);
#9650=ORIENTED_EDGE('',*,*,#6532,.F.);
#9651=ORIENTED_EDGE('',*,*,#6495,.F.);
#9652=ORIENTED_EDGE('',*,*,#6507,.F.);
#9653=ORIENTED_EDGE('',*,*,#6493,.F.);
#9654=ORIENTED_EDGE('',*,*,#6531,.F.);
#9655=ORIENTED_EDGE('',*,*,#6512,.F.);
#9656=ORIENTED_EDGE('',*,*,#6508,.F.);
#9657=ORIENTED_EDGE('',*,*,#6485,.F.);
#9658=ORIENTED_EDGE('',*,*,#6527,.F.);
#9659=ORIENTED_EDGE('',*,*,#6489,.F.);
#9660=ORIENTED_EDGE('',*,*,#6506,.F.);
#9661=ORIENTED_EDGE('',*,*,#6545,.T.);
#9662=ORIENTED_EDGE('',*,*,#6542,.T.);
#9663=ORIENTED_EDGE('',*,*,#6546,.T.);
#9664=ORIENTED_EDGE('',*,*,#6511,.T.);
#9665=ORIENTED_EDGE('',*,*,#6546,.F.);
#9666=ORIENTED_EDGE('',*,*,#6541,.T.);
#9667=ORIENTED_EDGE('',*,*,#6547,.T.);
#9668=ORIENTED_EDGE('',*,*,#6526,.T.);
#9669=ORIENTED_EDGE('',*,*,#6545,.F.);
#9670=ORIENTED_EDGE('',*,*,#6525,.T.);
#9671=ORIENTED_EDGE('',*,*,#6548,.T.);
#9672=ORIENTED_EDGE('',*,*,#6543,.T.);
#9673=ORIENTED_EDGE('',*,*,#6547,.F.);
#9674=ORIENTED_EDGE('',*,*,#6544,.T.);
#9675=ORIENTED_EDGE('',*,*,#6548,.F.);
#9676=ORIENTED_EDGE('',*,*,#6524,.T.);
#10154=CYLINDRICAL_SURFACE('',#11608,4.);
#10155=CYLINDRICAL_SURFACE('',#11611,4.);
#10156=CYLINDRICAL_SURFACE('',#11614,2.5);
#10157=CYLINDRICAL_SURFACE('',#11617,2.5);
#10158=CYLINDRICAL_SURFACE('',#11620,2.5);
#10159=CYLINDRICAL_SURFACE('',#11623,2.5);
#10160=CYLINDRICAL_SURFACE('',#11626,3.);
#10161=CYLINDRICAL_SURFACE('',#11629,2.99999999999999);
#10162=CYLINDRICAL_SURFACE('',#11632,3.);
#10163=CYLINDRICAL_SURFACE('',#11635,3.);
#10164=CYLINDRICAL_SURFACE('',#11638,3.);
#10165=CYLINDRICAL_SURFACE('',#11641,3.);
#10166=CYLINDRICAL_SURFACE('',#11644,17.5);
#10167=CYLINDRICAL_SURFACE('',#11675,17.5);
#10168=CYLINDRICAL_SURFACE('',#11676,2.50000000000001);
#10169=CYLINDRICAL_SURFACE('',#11677,2.5);
#10170=CYLINDRICAL_SURFACE('',#11678,17.5);
#10171=CYLINDRICAL_SURFACE('',#11679,2.50000000000001);
#10172=CYLINDRICAL_SURFACE('',#11680,2.5);
#10173=CYLINDRICAL_SURFACE('',#11681,3.);
#10174=CYLINDRICAL_SURFACE('',#11684,3.);
#10175=CYLINDRICAL_SURFACE('',#11686,3.);
#10176=CYLINDRICAL_SURFACE('',#11688,3.);
#10697=ADVANCED_FACE('',(#2052),#10154,.F.);
#10698=ADVANCED_FACE('',(#2053),#10155,.F.);
#10699=ADVANCED_FACE('',(#2054),#10156,.F.);
#10700=ADVANCED_FACE('',(#2055),#10157,.F.);
#10701=ADVANCED_FACE('',(#2056),#10158,.F.);
#10702=ADVANCED_FACE('',(#2057),#10159,.F.);
#10703=ADVANCED_FACE('',(#2058),#10160,.F.);
#10704=ADVANCED_FACE('',(#2059),#10161,.F.);
#10705=ADVANCED_FACE('',(#2060),#10162,.F.);
#10706=ADVANCED_FACE('',(#2061),#10163,.F.);
#10707=ADVANCED_FACE('',(#2062),#10164,.F.);
#10708=ADVANCED_FACE('',(#2063),#10165,.F.);
#10709=ADVANCED_FACE('',(#2064),#10166,.F.);
#10710=ADVANCED_FACE('',(#2065),#1509,.T.);
#10711=ADVANCED_FACE('',(#2066),#1510,.T.);
#10712=ADVANCED_FACE('',(#2067),#1511,.T.);
#10713=ADVANCED_FACE('',(#2068),#1512,.T.);
#10714=ADVANCED_FACE('',(#2069),#1513,.T.);
#10715=ADVANCED_FACE('',(#2070,#1407,#1408),#1514,.F.);
#10716=ADVANCED_FACE('',(#2071),#1515,.T.);
#10717=ADVANCED_FACE('',(#2072,#1409,#1410),#1516,.F.);
#10718=ADVANCED_FACE('',(#2073),#1517,.F.);
#10719=ADVANCED_FACE('',(#2074,#1411),#1518,.F.);
#10720=ADVANCED_FACE('',(#2075,#1412,#1413),#1519,.T.);
#10721=ADVANCED_FACE('',(#2076,#1414),#1520,.T.);
#10722=ADVANCED_FACE('',(#2077,#1415,#1416),#1521,.T.);
#10723=ADVANCED_FACE('',(#2078),#1522,.T.);
#10724=ADVANCED_FACE('',(#2079,#1417,#1418,#1419,#1420,#1421,#1422,#1423,
#1424),#1523,.F.);
#10725=ADVANCED_FACE('',(#2080,#1425,#1426,#1427,#1428,#1429,#1430,#1431,
#1432),#1524,.T.);
#10726=ADVANCED_FACE('',(#2081),#10167,.F.);
#10727=ADVANCED_FACE('',(#2082),#10168,.F.);
#10728=ADVANCED_FACE('',(#2083),#10169,.F.);
#10729=ADVANCED_FACE('',(#2084),#10170,.F.);
#10730=ADVANCED_FACE('',(#2085),#10171,.F.);
#10731=ADVANCED_FACE('',(#2086),#10172,.F.);
#10732=ADVANCED_FACE('',(#2087),#10173,.T.);
#10733=ADVANCED_FACE('',(#2088),#10174,.T.);
#10734=ADVANCED_FACE('',(#2089),#10175,.T.);
#10735=ADVANCED_FACE('',(#2090),#10176,.T.);
#10823=CLOSED_SHELL('',(#10697,#10698,#10699,#10700,#10701,#10702,#10703,
#10704,#10705,#10706,#10707,#10708,#10709,#10710,#10711,#10712,#10713,#10714,
#10715,#10716,#10717,#10718,#10719,#10720,#10721,#10722,#10723,#10724,#10725,
#10726,#10727,#10728,#10729,#10730,#10731,#10732,#10733,#10734,#10735));
#11607=AXIS2_PLACEMENT_3D('',#37221,#13306,#13307);
#11608=AXIS2_PLACEMENT_3D('',#37222,#13308,#13309);
#11609=AXIS2_PLACEMENT_3D('',#37224,#13310,#13311);
#11610=AXIS2_PLACEMENT_3D('',#37227,#13313,#13314);
#11611=AXIS2_PLACEMENT_3D('',#37228,#13315,#13316);
#11612=AXIS2_PLACEMENT_3D('',#37230,#13317,#13318);
#11613=AXIS2_PLACEMENT_3D('',#37233,#13320,#13321);
#11614=AXIS2_PLACEMENT_3D('',#37234,#13322,#13323);
#11615=AXIS2_PLACEMENT_3D('',#37236,#13324,#13325);
#11616=AXIS2_PLACEMENT_3D('',#37239,#13327,#13328);
#11617=AXIS2_PLACEMENT_3D('',#37240,#13329,#13330);
#11618=AXIS2_PLACEMENT_3D('',#37242,#13331,#13332);
#11619=AXIS2_PLACEMENT_3D('',#37245,#13334,#13335);
#11620=AXIS2_PLACEMENT_3D('',#37246,#13336,#13337);
#11621=AXIS2_PLACEMENT_3D('',#37248,#13338,#13339);
#11622=AXIS2_PLACEMENT_3D('',#37251,#13341,#13342);
#11623=AXIS2_PLACEMENT_3D('',#37252,#13343,#13344);
#11624=AXIS2_PLACEMENT_3D('',#37254,#13345,#13346);
#11625=AXIS2_PLACEMENT_3D('',#37257,#13348,#13349);
#11626=AXIS2_PLACEMENT_3D('',#37258,#13350,#13351);
#11627=AXIS2_PLACEMENT_3D('',#37260,#13352,#13353);
#11628=AXIS2_PLACEMENT_3D('',#37263,#13355,#13356);
#11629=AXIS2_PLACEMENT_3D('',#37264,#13357,#13358);
#11630=AXIS2_PLACEMENT_3D('',#37266,#13359,#13360);
#11631=AXIS2_PLACEMENT_3D('',#37269,#13362,#13363);
#11632=AXIS2_PLACEMENT_3D('',#37270,#13364,#13365);
#11633=AXIS2_PLACEMENT_3D('',#37272,#13366,#13367);
#11634=AXIS2_PLACEMENT_3D('',#37275,#13369,#13370);
#11635=AXIS2_PLACEMENT_3D('',#37276,#13371,#13372);
#11636=AXIS2_PLACEMENT_3D('',#37278,#13373,#13374);
#11637=AXIS2_PLACEMENT_3D('',#37281,#13376,#13377);
#11638=AXIS2_PLACEMENT_3D('',#37282,#13378,#13379);
#11639=AXIS2_PLACEMENT_3D('',#37284,#13380,#13381);
#11640=AXIS2_PLACEMENT_3D('',#37287,#13383,#13384);
#11641=AXIS2_PLACEMENT_3D('',#37288,#13385,#13386);
#11642=AXIS2_PLACEMENT_3D('',#37290,#13387,#13388);
#11643=AXIS2_PLACEMENT_3D('',#37293,#13390,#13391);
#11644=AXIS2_PLACEMENT_3D('',#37294,#13392,#13393);
#11645=AXIS2_PLACEMENT_3D('',#37296,#13394,#13395);
#11646=AXIS2_PLACEMENT_3D('',#37299,#13397,#13398);
#11647=AXIS2_PLACEMENT_3D('',#37300,#13399,#13400);
#11648=AXIS2_PLACEMENT_3D('',#37317,#13409,#13410);
#11649=AXIS2_PLACEMENT_3D('',#37326,#13415,#13416);
#11650=AXIS2_PLACEMENT_3D('',#37335,#13421,#13422);
#11651=AXIS2_PLACEMENT_3D('',#37344,#13427,#13428);
#11652=AXIS2_PLACEMENT_3D('',#37353,#13433,#13434);
#11653=AXIS2_PLACEMENT_3D('',#37356,#13436,#13437);
#11654=AXIS2_PLACEMENT_3D('',#37357,#13438,#13439);
#11655=AXIS2_PLACEMENT_3D('',#37359,#13440,#13441);
#11656=AXIS2_PLACEMENT_3D('',#37365,#13445,#13446);
#11657=AXIS2_PLACEMENT_3D('',#37379,#13454,#13455);
#11658=AXIS2_PLACEMENT_3D('',#37382,#13457,#13458);
#11659=AXIS2_PLACEMENT_3D('',#37383,#13459,#13460);
#11660=AXIS2_PLACEMENT_3D('',#37384,#13461,#13462);
#11661=AXIS2_PLACEMENT_3D('',#37388,#13465,#13466);
#11662=AXIS2_PLACEMENT_3D('',#37390,#13468,#13469);
#11663=AXIS2_PLACEMENT_3D('',#37392,#13471,#13472);
#11664=AXIS2_PLACEMENT_3D('',#37393,#13473,#13474);
#11665=AXIS2_PLACEMENT_3D('',#37399,#13478,#13479);
#11666=AXIS2_PLACEMENT_3D('',#37400,#13480,#13481);
#11667=AXIS2_PLACEMENT_3D('',#37401,#13482,#13483);
#11668=AXIS2_PLACEMENT_3D('',#37405,#13486,#13487);
#11669=AXIS2_PLACEMENT_3D('',#37406,#13488,#13489);
#11670=AXIS2_PLACEMENT_3D('',#37407,#13490,#13491);
#11671=AXIS2_PLACEMENT_3D('',#37408,#13492,#13493);
#11672=AXIS2_PLACEMENT_3D('',#37412,#13496,#13497);
#11673=AXIS2_PLACEMENT_3D('',#37414,#13499,#13500);
#11674=AXIS2_PLACEMENT_3D('',#37415,#13501,#13502);
#11675=AXIS2_PLACEMENT_3D('',#37424,#13507,#13508);
#11676=AXIS2_PLACEMENT_3D('',#37425,#13509,#13510);
#11677=AXIS2_PLACEMENT_3D('',#37426,#13511,#13512);
#11678=AXIS2_PLACEMENT_3D('',#37427,#13513,#13514);
#11679=AXIS2_PLACEMENT_3D('',#37428,#13515,#13516);
#11680=AXIS2_PLACEMENT_3D('',#37429,#13517,#13518);
#11681=AXIS2_PLACEMENT_3D('',#37430,#13519,#13520);
#11682=AXIS2_PLACEMENT_3D('',#37431,#13521,#13522);
#11683=AXIS2_PLACEMENT_3D('',#37432,#13523,#13524);
#11684=AXIS2_PLACEMENT_3D('',#37433,#13525,#13526);
#11685=AXIS2_PLACEMENT_3D('',#37434,#13527,#13528);
#11686=AXIS2_PLACEMENT_3D('',#37435,#13529,#13530);
#11687=AXIS2_PLACEMENT_3D('',#37436,#13531,#13532);
#11688=AXIS2_PLACEMENT_3D('',#37437,#13533,#13534);
#13306=DIRECTION('axis',(0.,0.,1.));
#13307=DIRECTION('refdir',(1.,0.,0.));
#13308=DIRECTION('center_axis',(0.,1.,0.));
#13309=DIRECTION('ref_axis',(0.,0.,1.));
#13310=DIRECTION('center_axis',(0.,1.,0.));
#13311=DIRECTION('ref_axis',(0.,0.,-1.));
#13312=DIRECTION('',(0.,1.,0.));
#13313=DIRECTION('center_axis',(0.,1.,0.));
#13314=DIRECTION('ref_axis',(0.,0.,1.));
#13315=DIRECTION('center_axis',(0.,0.,-1.));
#13316=DIRECTION('ref_axis',(-1.,0.,0.));
#13317=DIRECTION('center_axis',(0.,0.,-1.));
#13318=DIRECTION('ref_axis',(-1.,0.,0.));
#13319=DIRECTION('',(0.,0.,-1.));
#13320=DIRECTION('center_axis',(0.,0.,-1.));
#13321=DIRECTION('ref_axis',(-1.,0.,0.));
#13322=DIRECTION('center_axis',(1.,0.,0.));
#13323=DIRECTION('ref_axis',(0.,0.,1.));
#13324=DIRECTION('center_axis',(1.,0.,0.));
#13325=DIRECTION('ref_axis',(0.,0.,-1.));
#13326=DIRECTION('',(1.,0.,0.));
#13327=DIRECTION('center_axis',(-1.,0.,0.));
#13328=DIRECTION('ref_axis',(0.,0.,1.));
#13329=DIRECTION('center_axis',(1.,0.,0.));
#13330=DIRECTION('ref_axis',(0.,0.,1.));
#13331=DIRECTION('center_axis',(1.,0.,0.));
#13332=DIRECTION('ref_axis',(0.,0.,-1.));
#13333=DIRECTION('',(1.,0.,0.));
#13334=DIRECTION('center_axis',(-1.,0.,0.));
#13335=DIRECTION('ref_axis',(0.,0.,1.));
#13336=DIRECTION('center_axis',(1.,0.,0.));
#13337=DIRECTION('ref_axis',(0.,0.,1.));
#13338=DIRECTION('center_axis',(-1.,0.,0.));
#13339=DIRECTION('ref_axis',(0.,0.,1.));
#13340=DIRECTION('',(1.,0.,0.));
#13341=DIRECTION('center_axis',(-1.,0.,0.));
#13342=DIRECTION('ref_axis',(0.,0.,1.));
#13343=DIRECTION('center_axis',(1.,0.,0.));
#13344=DIRECTION('ref_axis',(0.,0.,1.));
#13345=DIRECTION('center_axis',(-1.,0.,0.));
#13346=DIRECTION('ref_axis',(0.,0.,1.));
#13347=DIRECTION('',(1.,0.,0.));
#13348=DIRECTION('center_axis',(-1.,0.,0.));
#13349=DIRECTION('ref_axis',(0.,0.,1.));
#13350=DIRECTION('center_axis',(0.,0.,-1.));
#13351=DIRECTION('ref_axis',(1.,0.,0.));
#13352=DIRECTION('center_axis',(0.,0.,1.));
#13353=DIRECTION('ref_axis',(1.,0.,0.));
#13354=DIRECTION('',(0.,0.,-1.));
#13355=DIRECTION('center_axis',(0.,0.,1.));
#13356=DIRECTION('ref_axis',(1.,0.,0.));
#13357=DIRECTION('center_axis',(0.,0.,-1.));
#13358=DIRECTION('ref_axis',(1.,0.,0.));
#13359=DIRECTION('center_axis',(0.,0.,1.));
#13360=DIRECTION('ref_axis',(1.,0.,0.));
#13361=DIRECTION('',(0.,0.,-1.));
#13362=DIRECTION('center_axis',(0.,0.,1.));
#13363=DIRECTION('ref_axis',(1.,0.,0.));
#13364=DIRECTION('center_axis',(0.,0.,-1.));
#13365=DIRECTION('ref_axis',(1.,0.,0.));
#13366=DIRECTION('center_axis',(0.,0.,1.));
#13367=DIRECTION('ref_axis',(1.,0.,0.));
#13368=DIRECTION('',(0.,0.,-1.));
#13369=DIRECTION('center_axis',(0.,0.,1.));
#13370=DIRECTION('ref_axis',(1.,0.,0.));
#13371=DIRECTION('center_axis',(0.,0.,-1.));
#13372=DIRECTION('ref_axis',(1.,0.,0.));
#13373=DIRECTION('center_axis',(0.,0.,1.));
#13374=DIRECTION('ref_axis',(1.,0.,0.));
#13375=DIRECTION('',(0.,0.,-1.));
#13376=DIRECTION('center_axis',(0.,0.,1.));
#13377=DIRECTION('ref_axis',(1.,0.,0.));
#13378=DIRECTION('center_axis',(0.,0.,-1.));
#13379=DIRECTION('ref_axis',(1.,0.,0.));
#13380=DIRECTION('center_axis',(0.,0.,1.));
#13381=DIRECTION('ref_axis',(1.,0.,0.));
#13382=DIRECTION('',(0.,0.,-1.));
#13383=DIRECTION('center_axis',(0.,0.,1.));
#13384=DIRECTION('ref_axis',(1.,0.,0.));
#13385=DIRECTION('center_axis',(0.,0.,-1.));
#13386=DIRECTION('ref_axis',(1.,0.,0.));
#13387=DIRECTION('center_axis',(0.,0.,1.));
#13388=DIRECTION('ref_axis',(1.,0.,0.));
#13389=DIRECTION('',(0.,0.,-1.));
#13390=DIRECTION('center_axis',(0.,0.,1.));
#13391=DIRECTION('ref_axis',(1.,0.,0.));
#13392=DIRECTION('center_axis',(0.,0.,-1.));
#13393=DIRECTION('ref_axis',(1.,0.,0.));
#13394=DIRECTION('center_axis',(0.,0.,1.));
#13395=DIRECTION('ref_axis',(1.,0.,0.));
#13396=DIRECTION('',(0.,0.,-1.));
#13397=DIRECTION('center_axis',(0.,0.,1.));
#13398=DIRECTION('ref_axis',(1.,0.,0.));
#13399=DIRECTION('center_axis',(0.,0.,1.));
#13400=DIRECTION('ref_axis',(-1.,0.,0.));
#13401=DIRECTION('',(1.,0.,0.));
#13402=DIRECTION('',(0.,-1.,0.));
#13403=DIRECTION('',(-1.,0.,0.));
#13404=DIRECTION('',(0.,1.,0.));
#13405=DIRECTION('',(1.,0.,0.));
#13406=DIRECTION('',(0.,1.,0.));
#13407=DIRECTION('',(-1.,0.,0.));
#13408=DIRECTION('',(0.,-1.,0.));
#13409=DIRECTION('center_axis',(0.,0.,1.));
#13410=DIRECTION('ref_axis',(-1.,0.,0.));
#13411=DIRECTION('',(-1.,0.,0.));
#13412=DIRECTION('',(0.,1.,0.));
#13413=DIRECTION('',(1.,0.,0.));
#13414=DIRECTION('',(0.,1.,0.));
#13415=DIRECTION('center_axis',(0.,0.,1.));
#13416=DIRECTION('ref_axis',(-1.,0.,0.));
#13417=DIRECTION('',(1.,0.,0.));
#13418=DIRECTION('',(0.,1.,0.));
#13419=DIRECTION('',(-1.,0.,0.));
#13420=DIRECTION('',(0.,1.,0.));
#13421=DIRECTION('center_axis',(0.,0.,1.));
#13422=DIRECTION('ref_axis',(-1.,0.,0.));
#13423=DIRECTION('',(1.,0.,0.));
#13424=DIRECTION('',(0.,-1.,0.));
#13425=DIRECTION('',(-1.,0.,0.));
#13426=DIRECTION('',(0.,-1.,0.));
#13427=DIRECTION('center_axis',(0.,0.,1.));
#13428=DIRECTION('ref_axis',(-1.,0.,0.));
#13429=DIRECTION('',(-1.,0.,0.));
#13430=DIRECTION('',(0.,-1.,0.));
#13431=DIRECTION('',(1.,0.,0.));
#13432=DIRECTION('',(0.,-1.,0.));
#13433=DIRECTION('center_axis',(-1.,0.,0.));
#13434=DIRECTION('ref_axis',(0.,0.,-1.));
#13435=DIRECTION('',(0.,0.,1.));
#13436=DIRECTION('center_axis',(-1.,0.,0.));
#13437=DIRECTION('ref_axis',(0.,0.,1.));
#13438=DIRECTION('center_axis',(-1.,0.,0.));
#13439=DIRECTION('ref_axis',(0.,0.,1.));
#13440=DIRECTION('center_axis',(-1.,0.,0.));
#13441=DIRECTION('ref_axis',(0.,0.,1.));
#13442=DIRECTION('',(0.,1.,0.));
#13443=DIRECTION('',(0.,0.,1.));
#13444=DIRECTION('',(0.,-1.,0.));
#13445=DIRECTION('center_axis',(0.,0.,1.));
#13446=DIRECTION('ref_axis',(-1.,0.,0.));
#13447=DIRECTION('',(-1.,0.,0.));
#13448=DIRECTION('',(0.,1.,0.));
#13449=DIRECTION('',(1.,-1.33440267382831E-16,0.));
#13450=DIRECTION('',(0.,-1.,0.));
#13451=DIRECTION('',(-1.,0.,0.));
#13452=DIRECTION('',(0.,-1.,0.));
#13453=DIRECTION('',(1.,0.,0.));
#13454=DIRECTION('center_axis',(1.,0.,0.));
#13455=DIRECTION('ref_axis',(0.,0.,1.));
#13456=DIRECTION('',(0.,0.,1.));
#13457=DIRECTION('center_axis',(-1.,0.,0.));
#13458=DIRECTION('ref_axis',(0.,0.,1.));
#13459=DIRECTION('center_axis',(-1.,0.,0.));
#13460=DIRECTION('ref_axis',(0.,0.,1.));
#13461=DIRECTION('center_axis',(-1.,0.,0.));
#13462=DIRECTION('ref_axis',(0.,0.,1.));
#13463=DIRECTION('',(0.,0.,1.));
#13464=DIRECTION('',(0.,1.,0.));
#13465=DIRECTION('center_axis',(0.,1.,0.));
#13466=DIRECTION('ref_axis',(0.,0.,-1.));
#13467=DIRECTION('',(-1.,0.,0.));
#13468=DIRECTION('center_axis',(0.,-1.,0.));
#13469=DIRECTION('ref_axis',(0.,0.,1.));
#13470=DIRECTION('',(1.,0.,0.));
#13471=DIRECTION('center_axis',(-1.,0.,0.));
#13472=DIRECTION('ref_axis',(0.,0.,-1.));
#13473=DIRECTION('center_axis',(1.,0.,0.));
#13474=DIRECTION('ref_axis',(0.,0.,-1.));
#13475=DIRECTION('',(0.,0.,1.));
#13476=DIRECTION('',(0.,1.,0.));
#13477=DIRECTION('',(0.,0.,1.));
#13478=DIRECTION('center_axis',(1.,0.,0.));
#13479=DIRECTION('ref_axis',(0.,0.,-1.));
#13480=DIRECTION('center_axis',(1.,0.,0.));
#13481=DIRECTION('ref_axis',(0.,0.,-1.));
#13482=DIRECTION('center_axis',(0.,-1.,0.));
#13483=DIRECTION('ref_axis',(0.,0.,1.));
#13484=DIRECTION('',(0.,0.,1.));
#13485=DIRECTION('',(-1.,0.,0.));
#13486=DIRECTION('center_axis',(1.,0.,0.));
#13487=DIRECTION('ref_axis',(0.,0.,1.));
#13488=DIRECTION('center_axis',(-1.,0.,0.));
#13489=DIRECTION('ref_axis',(0.,0.,1.));
#13490=DIRECTION('center_axis',(-1.,0.,0.));
#13491=DIRECTION('ref_axis',(0.,0.,1.));
#13492=DIRECTION('center_axis',(-1.,0.,0.));
#13493=DIRECTION('ref_axis',(0.,0.,1.));
#13494=DIRECTION('',(0.,0.,1.));
#13495=DIRECTION('',(0.,-1.,0.));
#13496=DIRECTION('center_axis',(1.33440267382831E-16,1.,0.));
#13497=DIRECTION('ref_axis',(-1.,1.33440267382831E-16,0.));
#13498=DIRECTION('',(1.,-1.33440267382831E-16,0.));
#13499=DIRECTION('center_axis',(0.,0.,-1.));
#13500=DIRECTION('ref_axis',(1.,0.,0.));
#13501=DIRECTION('center_axis',(0.,0.,-1.));
#13502=DIRECTION('ref_axis',(1.,0.,0.));
#13503=DIRECTION('',(-1.,0.,0.));
#13504=DIRECTION('',(0.,1.,0.));
#13505=DIRECTION('',(1.,0.,0.));
#13506=DIRECTION('',(0.,-1.,0.));
#13507=DIRECTION('center_axis',(1.,0.,0.));
#13508=DIRECTION('ref_axis',(0.,1.22464679914735E-16,-1.));
#13509=DIRECTION('center_axis',(1.,0.,0.));
#13510=DIRECTION('ref_axis',(0.,1.22464679914735E-16,-1.));
#13511=DIRECTION('center_axis',(1.,0.,0.));
#13512=DIRECTION('ref_axis',(0.,1.22464679914735E-16,-1.));
#13513=DIRECTION('center_axis',(1.,0.,0.));
#13514=DIRECTION('ref_axis',(0.,1.22464679914735E-16,-1.));
#13515=DIRECTION('center_axis',(1.,0.,0.));
#13516=DIRECTION('ref_axis',(0.,1.22464679914735E-16,-1.));
#13517=DIRECTION('center_axis',(1.,0.,0.));
#13518=DIRECTION('ref_axis',(0.,1.22464679914735E-16,-1.));
#13519=DIRECTION('center_axis',(0.,-1.,0.));
#13520=DIRECTION('ref_axis',(0.,0.,1.));
#13521=DIRECTION('center_axis',(0.707106781186549,0.707106781186546,-1.57296168257423E-15));
#13522=DIRECTION('ref_axis',(0.707106781186546,-0.707106781186549,9.32138197837028E-14));
#13523=DIRECTION('center_axis',(0.707106781186548,-0.707106781186548,0.));
#13524=DIRECTION('ref_axis',(0.707106781186548,0.707106781186548,4.73150009852597E-13));
#13525=DIRECTION('center_axis',(1.,0.,0.));
#13526=DIRECTION('ref_axis',(0.,0.,1.));
#13527=DIRECTION('center_axis',(0.707106781186548,0.707106781186548,0.));
#13528=DIRECTION('ref_axis',(0.707106781186548,-0.707106781186548,-1.54176894316072E-13));
#13529=DIRECTION('center_axis',(-1.,0.,0.));
#13530=DIRECTION('ref_axis',(0.,0.,-1.));
#13531=DIRECTION('center_axis',(0.707106781186552,-0.707106781186543,6.49701564541535E-15));
#13532=DIRECTION('ref_axis',(0.707106781186543,0.707106781186552,-3.8859613000266E-13));
#13533=DIRECTION('center_axis',(0.,1.,0.));
#13534=DIRECTION('ref_axis',(0.,0.,-1.));
#37221=CARTESIAN_POINT('',(0.,0.,0.));
#37222=CARTESIAN_POINT('Origin',(46.,55.1862915010152,2.));
#37223=CARTESIAN_POINT('',(46.,66.5,-2.));
#37224=CARTESIAN_POINT('Origin',(46.,66.5,2.));
#37225=CARTESIAN_POINT('',(46.,76.5,-2.));
#37226=CARTESIAN_POINT('',(46.,55.1862915010152,-2.));
#37227=CARTESIAN_POINT('Origin',(46.,76.5,2.));
#37228=CARTESIAN_POINT('Origin',(42.0000000000001,-56.5,14.5));
#37229=CARTESIAN_POINT('',(46.0000000000001,-56.5,-14.5));
#37230=CARTESIAN_POINT('Origin',(42.,-56.5,-14.5));
#37231=CARTESIAN_POINT('',(46.0000000000001,-56.5,-24.5));
#37232=CARTESIAN_POINT('',(46.0000000000001,-56.5,14.5));
#37233=CARTESIAN_POINT('Origin',(42.,-56.5,-24.5));
#37234=CARTESIAN_POINT('Origin',(-62.,46.68,-3.68653347947321));
#37235=CARTESIAN_POINT('',(52.,46.68,-6.18653347947322));
#37236=CARTESIAN_POINT('Origin',(52.,46.68,-3.68653347947321));
#37237=CARTESIAN_POINT('',(62.,46.68,-6.18653347947322));
#37238=CARTESIAN_POINT('',(-62.,46.68,-6.18653347947322));
#37239=CARTESIAN_POINT('Origin',(62.,46.68,-3.68653347947321));
#37240=CARTESIAN_POINT('Origin',(-62.,25.68,-3.68653347947321));
#37241=CARTESIAN_POINT('',(52.,25.68,-6.18653347947322));
#37242=CARTESIAN_POINT('Origin',(52.,25.68,-3.68653347947321));
#37243=CARTESIAN_POINT('',(62.,25.68,-6.18653347947322));
#37244=CARTESIAN_POINT('',(-62.,25.68,-6.18653347947322));
#37245=CARTESIAN_POINT('Origin',(62.,25.68,-3.68653347947321));
#37246=CARTESIAN_POINT('Origin',(-62.,46.68,-3.68653347947321));
#37247=CARTESIAN_POINT('',(-62.,46.68,-6.18653347947322));
#37248=CARTESIAN_POINT('Origin',(-62.,46.68,-3.68653347947321));
#37249=CARTESIAN_POINT('',(-52.,46.68,-6.18653347947322));
#37250=CARTESIAN_POINT('',(-62.,46.68,-6.18653347947322));
#37251=CARTESIAN_POINT('Origin',(-52.,46.68,-3.68653347947321));
#37252=CARTESIAN_POINT('Origin',(-62.,25.68,-3.68653347947321));
#37253=CARTESIAN_POINT('',(-62.,25.68,-6.18653347947322));
#37254=CARTESIAN_POINT('Origin',(-62.,25.68,-3.68653347947321));
#37255=CARTESIAN_POINT('',(-52.,25.68,-6.18653347947322));
#37256=CARTESIAN_POINT('',(-62.,25.68,-6.18653347947322));
#37257=CARTESIAN_POINT('Origin',(-52.,25.68,-3.68653347947321));
#37258=CARTESIAN_POINT('Origin',(-26.3106350946109,-8.00000000000001,-14.5));
#37259=CARTESIAN_POINT('',(-29.3106350946109,-8.00000000000001,-14.5));
#37260=CARTESIAN_POINT('Origin',(-26.3106350946109,-8.00000000000001,-14.5));
#37261=CARTESIAN_POINT('',(-29.3106350946109,-8.00000000000001,-24.5));
#37262=CARTESIAN_POINT('',(-29.3106350946109,-8.00000000000001,-14.5));
#37263=CARTESIAN_POINT('Origin',(-26.3106350946109,-8.00000000000001,-24.5));
#37264=CARTESIAN_POINT('Origin',(-26.3106350946109,-33.,-14.5));
#37265=CARTESIAN_POINT('',(-29.3106350946109,-33.,-14.5));
#37266=CARTESIAN_POINT('Origin',(-26.3106350946109,-33.,-14.5));
#37267=CARTESIAN_POINT('',(-29.3106350946109,-33.,-24.5));
#37268=CARTESIAN_POINT('',(-29.3106350946109,-33.,-14.5));
#37269=CARTESIAN_POINT('Origin',(-26.3106350946109,-33.,-24.5));
#37270=CARTESIAN_POINT('Origin',(-4.66,-45.5,-14.5));
#37271=CARTESIAN_POINT('',(-7.66000000000001,-45.5,-14.5));
#37272=CARTESIAN_POINT('Origin',(-4.66,-45.5,-14.5));
#37273=CARTESIAN_POINT('',(-7.66000000000001,-45.5,-24.5));
#37274=CARTESIAN_POINT('',(-7.66000000000001,-45.5,-14.5));
#37275=CARTESIAN_POINT('Origin',(-4.66,-45.5,-24.5));
#37276=CARTESIAN_POINT('Origin',(16.990635094611,-33.,-14.5));
#37277=CARTESIAN_POINT('',(13.990635094611,-33.,-14.5));
#37278=CARTESIAN_POINT('Origin',(16.990635094611,-33.,-14.5));
#37279=CARTESIAN_POINT('',(13.990635094611,-33.,-24.5));
#37280=CARTESIAN_POINT('',(13.990635094611,-33.,-14.5));
#37281=CARTESIAN_POINT('Origin',(16.990635094611,-33.,-24.5));
#37282=CARTESIAN_POINT('Origin',(16.990635094611,-8.00000000000001,-14.5));
#37283=CARTESIAN_POINT('',(13.990635094611,-8.00000000000001,-14.5));
#37284=CARTESIAN_POINT('Origin',(16.990635094611,-8.00000000000001,-14.5));
#37285=CARTESIAN_POINT('',(13.990635094611,-8.00000000000001,-24.5));
#37286=CARTESIAN_POINT('',(13.990635094611,-8.00000000000001,-14.5));
#37287=CARTESIAN_POINT('Origin',(16.990635094611,-8.00000000000001,-24.5));
#37288=CARTESIAN_POINT('Origin',(-4.66,4.49999999999999,-14.5));
#37289=CARTESIAN_POINT('',(-7.66,4.49999999999999,-14.5));
#37290=CARTESIAN_POINT('Origin',(-4.66,4.49999999999999,-14.5));
#37291=CARTESIAN_POINT('',(-7.66,4.49999999999999,-24.5));
#37292=CARTESIAN_POINT('',(-7.66,4.49999999999999,-14.5));
#37293=CARTESIAN_POINT('Origin',(-4.66,4.49999999999999,-24.5));
#37294=CARTESIAN_POINT('Origin',(-4.66,-20.5,-14.5));
#37295=CARTESIAN_POINT('',(-22.16,-20.5,-14.5));
#37296=CARTESIAN_POINT('Origin',(-4.66,-20.5,-14.5));
#37297=CARTESIAN_POINT('',(-22.16,-20.5,-24.5));
#37298=CARTESIAN_POINT('',(-22.16,-20.5,-14.5));
#37299=CARTESIAN_POINT('Origin',(-4.66,-20.5,-24.5));
#37300=CARTESIAN_POINT('Origin',(0.,0.,14.5));
#37301=CARTESIAN_POINT('',(-61.9999999999999,59.68,14.5));
#37302=CARTESIAN_POINT('',(-51.9999999999999,59.68,14.5));
#37303=CARTESIAN_POINT('',(-61.9999999999999,59.68,14.5));
#37304=CARTESIAN_POINT('',(-51.9999999999999,66.5,14.5));
#37305=CARTESIAN_POINT('',(-51.9999999999999,-66.5,14.5));
#37306=CARTESIAN_POINT('',(52.0000000000001,66.5,14.5));
#37307=CARTESIAN_POINT('',(-51.9999999999999,66.5,14.5));
#37308=CARTESIAN_POINT('',(52.0000000000001,59.68,14.5));
#37309=CARTESIAN_POINT('',(52.0000000000001,-66.5,14.5));
#37310=CARTESIAN_POINT('',(62.0000000000001,59.68,14.5));
#37311=CARTESIAN_POINT('',(-61.9999999999999,59.68,14.5));
#37312=CARTESIAN_POINT('',(62.0000000000001,76.5,14.5));
#37313=CARTESIAN_POINT('',(62.0000000000001,-76.5,14.5));
#37314=CARTESIAN_POINT('',(-61.9999999999999,76.5,14.5));
#37315=CARTESIAN_POINT('',(-61.9999999999999,76.5,14.5));
#37316=CARTESIAN_POINT('',(-61.9999999999999,-76.5,14.5));
#37317=CARTESIAN_POINT('Origin',(0.,0.,14.5));
#37318=CARTESIAN_POINT('',(62.0000000000001,54.68,14.5));
#37319=CARTESIAN_POINT('',(52.0000000000001,54.68,14.5));
#37320=CARTESIAN_POINT('',(-61.9999999999999,54.68,14.5));
#37321=CARTESIAN_POINT('',(52.0000000000001,53.68,14.5));
#37322=CARTESIAN_POINT('',(52.0000000000001,-66.5,14.5));
#37323=CARTESIAN_POINT('',(62.0000000000001,53.68,14.5));
#37324=CARTESIAN_POINT('',(-61.9999999999999,53.68,14.5));
#37325=CARTESIAN_POINT('',(62.0000000000001,-76.5,14.5));
#37326=CARTESIAN_POINT('Origin',(0.,0.,14.5));
#37327=CARTESIAN_POINT('',(52.0000000000001,17.68,14.5));
#37328=CARTESIAN_POINT('',(62.0000000000001,17.68,14.5));
#37329=CARTESIAN_POINT('',(-61.9999999999999,17.68,14.5));
#37330=CARTESIAN_POINT('',(62.0000000000001,18.68,14.5));
#37331=CARTESIAN_POINT('',(62.0000000000001,-76.5,14.5));
#37332=CARTESIAN_POINT('',(52.0000000000001,18.68,14.5));
#37333=CARTESIAN_POINT('',(-61.9999999999999,18.68,14.5));
#37334=CARTESIAN_POINT('',(52.0000000000001,-66.5,14.5));
#37335=CARTESIAN_POINT('Origin',(0.,0.,14.5));
#37336=CARTESIAN_POINT('',(-61.9999999999999,17.68,14.5));
#37337=CARTESIAN_POINT('',(-51.9999999999999,17.68,14.5));
#37338=CARTESIAN_POINT('',(-61.9999999999999,17.68,14.5));
#37339=CARTESIAN_POINT('',(-51.9999999999999,18.68,14.5));
#37340=CARTESIAN_POINT('',(-51.9999999999999,-66.5,14.5));
#37341=CARTESIAN_POINT('',(-61.9999999999999,18.68,14.5));
#37342=CARTESIAN_POINT('',(-61.9999999999999,18.68,14.5));
#37343=CARTESIAN_POINT('',(-61.9999999999999,-76.5,14.5));
#37344=CARTESIAN_POINT('Origin',(0.,0.,14.5));
#37345=CARTESIAN_POINT('',(-51.9999999999999,54.68,14.5));
#37346=CARTESIAN_POINT('',(-61.9999999999999,54.68,14.5));
#37347=CARTESIAN_POINT('',(-61.9999999999999,54.68,14.5));
#37348=CARTESIAN_POINT('',(-61.9999999999999,53.68,14.5));
#37349=CARTESIAN_POINT('',(-61.9999999999999,-76.5,14.5));
#37350=CARTESIAN_POINT('',(-51.9999999999999,53.68,14.5));
#37351=CARTESIAN_POINT('',(-61.9999999999999,53.68,14.5));
#37352=CARTESIAN_POINT('',(-51.9999999999999,-66.5,14.5));
#37353=CARTESIAN_POINT('Origin',(62.,-76.5,-14.5));
#37354=CARTESIAN_POINT('',(62.,76.5,-21.5));
#37355=CARTESIAN_POINT('',(62.,76.5,-14.5));
#37356=CARTESIAN_POINT('Origin',(62.0000000000001,57.18,14.5));
#37357=CARTESIAN_POINT('Origin',(62.0000000000001,36.18,14.5));
#37358=CARTESIAN_POINT('',(62.0000000000001,12.68,14.5));
#37359=CARTESIAN_POINT('Origin',(62.0000000000001,15.18,14.5));
#37360=CARTESIAN_POINT('',(62.0000000000001,-76.5,14.5));
#37361=CARTESIAN_POINT('',(62.0000000000001,-76.5,14.5));
#37362=CARTESIAN_POINT('',(62.,-76.5,-21.5));
#37363=CARTESIAN_POINT('',(62.,-76.5,-14.5));
#37364=CARTESIAN_POINT('',(62.,-76.5,-21.5));
#37365=CARTESIAN_POINT('Origin',(0.,0.,14.5));
#37366=CARTESIAN_POINT('',(52.0000000000001,12.68,14.5));
#37367=CARTESIAN_POINT('',(-61.9999999999999,12.68,14.5));
#37368=CARTESIAN_POINT('',(52.0000000000001,-66.5,14.5));
#37369=CARTESIAN_POINT('',(52.0000000000001,-66.5,14.5));
#37370=CARTESIAN_POINT('',(-51.9999999999999,-66.5,14.5));
#37371=CARTESIAN_POINT('',(-51.9999999999999,-66.5,14.5));
#37372=CARTESIAN_POINT('',(-51.9999999999999,12.68,14.5));
#37373=CARTESIAN_POINT('',(-51.9999999999999,-66.5,14.5));
#37374=CARTESIAN_POINT('',(-61.9999999999999,12.68,14.5));
#37375=CARTESIAN_POINT('',(-61.9999999999999,12.68,14.5));
#37376=CARTESIAN_POINT('',(-61.9999999999999,-76.5,14.5));
#37377=CARTESIAN_POINT('',(-61.9999999999999,-76.5,14.5));
#37378=CARTESIAN_POINT('',(-61.9999999999999,-76.5,14.5));
#37379=CARTESIAN_POINT('Origin',(-62.,-76.5,-14.5));
#37380=CARTESIAN_POINT('',(-62.,-76.5,-21.5));
#37381=CARTESIAN_POINT('',(-62.,-76.5,-14.5));
#37382=CARTESIAN_POINT('Origin',(-61.9999999999999,15.18,14.5));
#37383=CARTESIAN_POINT('Origin',(-61.9999999999999,36.18,14.5));
#37384=CARTESIAN_POINT('Origin',(-61.9999999999999,57.18,14.5));
#37385=CARTESIAN_POINT('',(-62.,76.5,-21.5));
#37386=CARTESIAN_POINT('',(-62.,76.5,-14.5));
#37387=CARTESIAN_POINT('',(-62.,76.5,-21.5));
#37388=CARTESIAN_POINT('Origin',(-62.,-76.5,-14.5));
#37389=CARTESIAN_POINT('',(-62.,-76.5,-21.5));
#37390=CARTESIAN_POINT('Origin',(-62.,76.5,-14.5));
#37391=CARTESIAN_POINT('',(62.,76.5,-21.5));
#37392=CARTESIAN_POINT('Origin',(52.,-66.5,-14.5));
#37393=CARTESIAN_POINT('Origin',(52.0000000000001,57.18,14.5));
#37394=CARTESIAN_POINT('',(52.,66.5,-14.5));
#37395=CARTESIAN_POINT('',(52.,66.5,-14.5));
#37396=CARTESIAN_POINT('',(52.,-66.5,-14.5));
#37397=CARTESIAN_POINT('',(52.,-66.5,-14.5));
#37398=CARTESIAN_POINT('',(52.,-66.5,-14.5));
#37399=CARTESIAN_POINT('Origin',(52.0000000000001,15.18,14.5));
#37400=CARTESIAN_POINT('Origin',(52.0000000000001,36.18,14.5));
#37401=CARTESIAN_POINT('Origin',(-52.,66.5,-14.5));
#37402=CARTESIAN_POINT('',(-52.,66.5,-14.5));
#37403=CARTESIAN_POINT('',(-52.,66.5,-14.5));
#37404=CARTESIAN_POINT('',(-52.,66.5,-14.5));
#37405=CARTESIAN_POINT('Origin',(-52.,-66.5,-14.5));
#37406=CARTESIAN_POINT('Origin',(-51.9999999999999,57.18,14.5));
#37407=CARTESIAN_POINT('Origin',(-51.9999999999999,36.18,14.5));
#37408=CARTESIAN_POINT('Origin',(-51.9999999999999,15.18,14.5));
#37409=CARTESIAN_POINT('',(-52.,-66.5,-14.5));
#37410=CARTESIAN_POINT('',(-52.,-66.5,-14.5));
#37411=CARTESIAN_POINT('',(-52.,-66.5,-14.5));
#37412=CARTESIAN_POINT('Origin',(-52.,-66.5,-14.5));
#37413=CARTESIAN_POINT('',(-52.,-66.5,-14.5));
#37414=CARTESIAN_POINT('Origin',(0.,0.,-14.5));
#37415=CARTESIAN_POINT('Origin',(0.,0.,-24.5));
#37416=CARTESIAN_POINT('',(59.,73.5,-24.5));
#37417=CARTESIAN_POINT('',(-59.,73.5,-24.5));
#37418=CARTESIAN_POINT('',(-62.,73.5,-24.5));
#37419=CARTESIAN_POINT('',(59.,-73.5,-24.5));
#37420=CARTESIAN_POINT('',(59.,76.5,-24.5));
#37421=CARTESIAN_POINT('',(-59.,-73.5,-24.5));
#37422=CARTESIAN_POINT('',(62.,-73.5,-24.5));
#37423=CARTESIAN_POINT('',(-59.,-76.5,-24.5));
#37424=CARTESIAN_POINT('Origin',(-61.9999999999999,36.18,14.5));
#37425=CARTESIAN_POINT('Origin',(-61.9999999999999,15.18,14.5));
#37426=CARTESIAN_POINT('Origin',(-61.9999999999999,57.18,14.5));
#37427=CARTESIAN_POINT('Origin',(-61.9999999999999,36.18,14.5));
#37428=CARTESIAN_POINT('Origin',(-61.9999999999999,15.18,14.5));
#37429=CARTESIAN_POINT('Origin',(-61.9999999999999,57.18,14.5));
#37430=CARTESIAN_POINT('Origin',(59.,0.,-21.5));
#37431=CARTESIAN_POINT('Origin',(59.0000000000003,-73.5000000000003,-21.5000000000003));
#37432=CARTESIAN_POINT('Origin',(59.0000000000012,73.5000000000012,-21.5000000000012));
#37433=CARTESIAN_POINT('Origin',(4.93038065763132E-29,73.5,-21.5));
#37434=CARTESIAN_POINT('Origin',(-59.0000000000004,73.5000000000004,-21.5000000000004));
#37435=CARTESIAN_POINT('Origin',(4.93038065763132E-29,-73.5,-21.5));
#37436=CARTESIAN_POINT('Origin',(-59.000000000001,-73.500000000001,-21.500000000001));
#37437=CARTESIAN_POINT('Origin',(-59.,0.,-21.5));
#37859=UNCERTAINTY_MEASURE_WITH_UNIT(LENGTH_MEASURE(0.01),#37882,
'DISTANCE_ACCURACY_VALUE',
'Maximum model space distance between geometric entities at asserted c
onnectivities');
#37867=UNCERTAINTY_MEASURE_WITH_UNIT(LENGTH_MEASURE(0.01),#37882,
'DISTANCE_ACCURACY_VALUE',
'Maximum model space distance between geometric entities at asserted c
onnectivities');
#37873=(
GEOMETRIC_REPRESENTATION_CONTEXT(3)
GLOBAL_UNCERTAINTY_ASSIGNED_CONTEXT((#37859))
GLOBAL_UNIT_ASSIGNED_CONTEXT((#37882,#37884,#37885))
REPRESENTATION_CONTEXT('','3D')
);
#37881=(
GEOMETRIC_REPRESENTATION_CONTEXT(3)
GLOBAL_UNCERTAINTY_ASSIGNED_CONTEXT((#37867))
GLOBAL_UNIT_ASSIGNED_CONTEXT((#37882,#37884,#37885))
REPRESENTATION_CONTEXT('','3D')
);
#37882=(
LENGTH_UNIT()
NAMED_UNIT(*)
SI_UNIT(.MILLI.,.METRE.)
);
#37884=(
NAMED_UNIT(*)
PLANE_ANGLE_UNIT()
SI_UNIT($,.RADIAN.)
);
#37885=(
NAMED_UNIT(*)
SI_UNIT($,.STERADIAN.)
SOLID_ANGLE_UNIT()
);
#37891=SHAPE_DEFINITION_REPRESENTATION(#37904,#37958);
#37904=PRODUCT_DEFINITION_SHAPE('',$,#37972);
#37958=SHAPE_REPRESENTATION('',(#11607),#37873);
#37966=PRODUCT_DEFINITION_CONTEXT('part definition',#38007,'design');
#37972=PRODUCT_DEFINITION('PS06','Body_B',#37985,#37966);
#37985=PRODUCT_DEFINITION_FORMATION('',$,#38014);
#38007=APPLICATION_CONTEXT(
'Core Data for Automotive Mechanical Design Process');
#38008=PRODUCT_CONTEXT('part definition',#38007,'mechanical');
#38014=PRODUCT('PS06','Body_B',$,(#38008));
#38023=PRESENTATION_STYLE_ASSIGNMENT((#38025));
#38025=SURFACE_STYLE_USAGE(.BOTH.,#38027);
#38027=SURFACE_SIDE_STYLE('',(#38029));
#38029=SURFACE_STYLE_FILL_AREA(#38031);
#38031=FILL_AREA_STYLE('Opaque(202,209,238)',(#38033));
#38033=FILL_AREA_STYLE_COLOUR('Opaque(202,209,238)',#38035);
#38035=COLOUR_RGB('Opaque(202,209,238)', 0.66274510, 0.83137255, 0.94901961);
ENDSEC;
END-ISO-10303-21;
